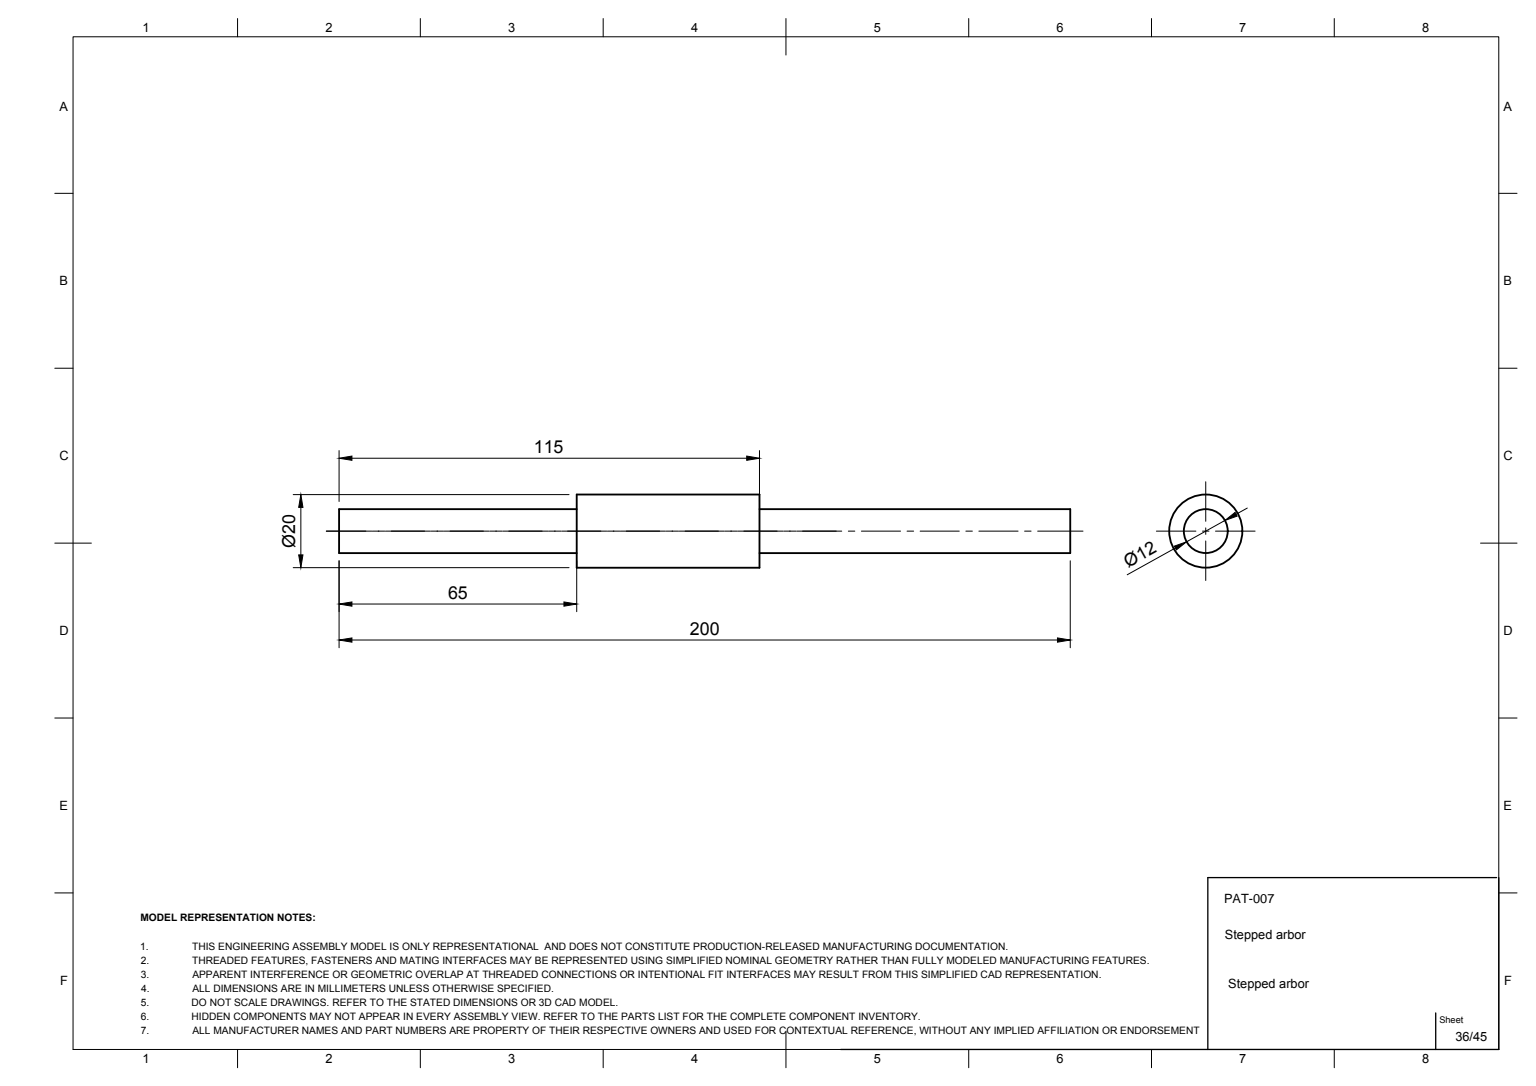
ISO-10303-21;
HEADER;
/* Generated by software containing ST-Developer
 * from STEP Tools, Inc. (www.steptools.com) 
 */

FILE_DESCRIPTION(
/* description */ ('Bearing friction torque test rig'),
/* implementation_level */ '2;1');

FILE_NAME(
/* name */ 'Stepped arbor.step',
/* time_stamp */ '2026-10-28T03:24:04-07:00',
/* author */ (''),
/* organization */ (''),
/* preprocessor_version */ 'ST-DEVELOPER v20.2',
/* originating_system */ 'Autodesk Translation Framework v15.17.0.0',
/* authorisation */ '');

FILE_SCHEMA (('AUTOMOTIVE_DESIGN { 1 0 10303 214 3 1 1 }'));
ENDSEC;

DATA;
#10=MECHANICAL_DESIGN_GEOMETRIC_PRESENTATION_REPRESENTATION('',(#582),#14822);
#489=SHAPE_REPRESENTATION_RELATIONSHIP('SRR','None',#15031,#528);
#528=ADVANCED_BREP_SHAPE_REPRESENTATION('',(#633),#14811);
#582=STYLED_ITEM('',(#15277),#633);
#633=MANIFOLD_SOLID_BREP('Body1',#7701);
#834=FACE_BOUND('',#2109,.T.);
#835=FACE_BOUND('',#2111,.T.);
#1057=PLANE('',#8995);
#1058=PLANE('',#8999);
#1059=PLANE('',#9003);
#1060=PLANE('',#9004);
#1468=FACE_OUTER_BOUND('',#2103,.T.);
#1469=FACE_OUTER_BOUND('',#2104,.T.);
#1470=FACE_OUTER_BOUND('',#2105,.T.);
#1471=FACE_OUTER_BOUND('',#2106,.T.);
#1472=FACE_OUTER_BOUND('',#2107,.T.);
#1473=FACE_OUTER_BOUND('',#2108,.T.);
#1474=FACE_OUTER_BOUND('',#2110,.T.);
#2103=EDGE_LOOP('',(#6738,#6739,#6740,#6741));
#2104=EDGE_LOOP('',(#6742));
#2105=EDGE_LOOP('',(#6743,#6744,#6745,#6746));
#2106=EDGE_LOOP('',(#6747));
#2107=EDGE_LOOP('',(#6748,#6749,#6750,#6751));
#2108=EDGE_LOOP('',(#6752));
#2109=EDGE_LOOP('',(#6753));
#2110=EDGE_LOOP('',(#6754));
#2111=EDGE_LOOP('',(#6755));
#2601=LINE('',#14102,#3045);
#2602=LINE('',#14109,#3046);
#2603=LINE('',#14116,#3047);
#3045=VECTOR('',#11252,0.6);
#3046=VECTOR('',#11261,0.6);
#3047=VECTOR('',#11270,1.);
#3482=CIRCLE('',#8993,0.6);
#3483=CIRCLE('',#8994,0.6);
#3484=CIRCLE('',#8997,0.6);
#3485=CIRCLE('',#8998,0.6);
#3486=CIRCLE('',#9001,1.);
#3487=CIRCLE('',#9002,1.);
#4097=VERTEX_POINT('',#14099);
#4098=VERTEX_POINT('',#14101);
#4099=VERTEX_POINT('',#14106);
#4100=VERTEX_POINT('',#14108);
#4101=VERTEX_POINT('',#14113);
#4102=VERTEX_POINT('',#14115);
#4995=EDGE_CURVE('',#4097,#4097,#3482,.T.);
#4996=EDGE_CURVE('',#4097,#4098,#2601,.T.);
#4997=EDGE_CURVE('',#4098,#4098,#3483,.T.);
#4998=EDGE_CURVE('',#4099,#4099,#3484,.T.);
#4999=EDGE_CURVE('',#4099,#4100,#2602,.T.);
#5000=EDGE_CURVE('',#4100,#4100,#3485,.T.);
#5001=EDGE_CURVE('',#4101,#4101,#3486,.T.);
#5002=EDGE_CURVE('',#4101,#4102,#2603,.T.);
#5003=EDGE_CURVE('',#4102,#4102,#3487,.T.);
#6738=ORIENTED_EDGE('',*,*,#4995,.F.);
#6739=ORIENTED_EDGE('',*,*,#4996,.T.);
#6740=ORIENTED_EDGE('',*,*,#4997,.F.);
#6741=ORIENTED_EDGE('',*,*,#4996,.F.);
#6742=ORIENTED_EDGE('',*,*,#4995,.T.);
#6743=ORIENTED_EDGE('',*,*,#4998,.F.);
#6744=ORIENTED_EDGE('',*,*,#4999,.T.);
#6745=ORIENTED_EDGE('',*,*,#5000,.T.);
#6746=ORIENTED_EDGE('',*,*,#4999,.F.);
#6747=ORIENTED_EDGE('',*,*,#5000,.F.);
#6748=ORIENTED_EDGE('',*,*,#5001,.F.);
#6749=ORIENTED_EDGE('',*,*,#5002,.T.);
#6750=ORIENTED_EDGE('',*,*,#5003,.T.);
#6751=ORIENTED_EDGE('',*,*,#5002,.F.);
#6752=ORIENTED_EDGE('',*,*,#5001,.T.);
#6753=ORIENTED_EDGE('',*,*,#4997,.T.);
#6754=ORIENTED_EDGE('',*,*,#5003,.F.);
#6755=ORIENTED_EDGE('',*,*,#4998,.T.);
#7178=CYLINDRICAL_SURFACE('',#8992,0.6);
#7179=CYLINDRICAL_SURFACE('',#8996,0.6);
#7180=CYLINDRICAL_SURFACE('',#9000,1.);
#7579=ADVANCED_FACE('',(#1468),#7178,.T.);
#7580=ADVANCED_FACE('',(#1469),#1057,.T.);
#7581=ADVANCED_FACE('',(#1470),#7179,.T.);
#7582=ADVANCED_FACE('',(#1471),#1058,.F.);
#7583=ADVANCED_FACE('',(#1472),#7180,.T.);
#7584=ADVANCED_FACE('',(#1473,#834),#1059,.T.);
#7585=ADVANCED_FACE('',(#1474,#835),#1060,.F.);
#7701=CLOSED_SHELL('',(#7579,#7580,#7581,#7582,#7583,#7584,#7585));
#8991=AXIS2_PLACEMENT_3D('',#14097,#11246,#11247);
#8992=AXIS2_PLACEMENT_3D('',#14098,#11248,#11249);
#8993=AXIS2_PLACEMENT_3D('',#14100,#11250,#11251);
#8994=AXIS2_PLACEMENT_3D('',#14103,#11253,#11254);
#8995=AXIS2_PLACEMENT_3D('',#14104,#11255,#11256);
#8996=AXIS2_PLACEMENT_3D('',#14105,#11257,#11258);
#8997=AXIS2_PLACEMENT_3D('',#14107,#11259,#11260);
#8998=AXIS2_PLACEMENT_3D('',#14110,#11262,#11263);
#8999=AXIS2_PLACEMENT_3D('',#14111,#11264,#11265);
#9000=AXIS2_PLACEMENT_3D('',#14112,#11266,#11267);
#9001=AXIS2_PLACEMENT_3D('',#14114,#11268,#11269);
#9002=AXIS2_PLACEMENT_3D('',#14117,#11271,#11272);
#9003=AXIS2_PLACEMENT_3D('',#14118,#11273,#11274);
#9004=AXIS2_PLACEMENT_3D('',#14119,#11275,#11276);
#11246=DIRECTION('axis',(0.,0.,1.));
#11247=DIRECTION('refdir',(1.,0.,0.));
#11248=DIRECTION('center_axis',(0.,1.,0.));
#11249=DIRECTION('ref_axis',(1.,0.,0.));
#11250=DIRECTION('center_axis',(0.,1.,0.));
#11251=DIRECTION('ref_axis',(1.,0.,0.));
#11252=DIRECTION('',(0.,-1.,0.));
#11253=DIRECTION('center_axis',(0.,-1.,0.));
#11254=DIRECTION('ref_axis',(1.,0.,0.));
#11255=DIRECTION('center_axis',(0.,1.,0.));
#11256=DIRECTION('ref_axis',(1.,0.,0.));
#11257=DIRECTION('center_axis',(0.,1.,0.));
#11258=DIRECTION('ref_axis',(1.,0.,0.));
#11259=DIRECTION('center_axis',(0.,1.,0.));
#11260=DIRECTION('ref_axis',(1.,0.,0.));
#11261=DIRECTION('',(0.,-1.,0.));
#11262=DIRECTION('center_axis',(0.,1.,0.));
#11263=DIRECTION('ref_axis',(1.,0.,0.));
#11264=DIRECTION('center_axis',(0.,1.,0.));
#11265=DIRECTION('ref_axis',(1.,0.,0.));
#11266=DIRECTION('center_axis',(0.,1.,0.));
#11267=DIRECTION('ref_axis',(1.,0.,0.));
#11268=DIRECTION('center_axis',(0.,1.,0.));
#11269=DIRECTION('ref_axis',(1.,0.,0.));
#11270=DIRECTION('',(0.,-1.,0.));
#11271=DIRECTION('center_axis',(0.,1.,0.));
#11272=DIRECTION('ref_axis',(1.,0.,0.));
#11273=DIRECTION('center_axis',(0.,1.,0.));
#11274=DIRECTION('ref_axis',(1.,0.,0.));
#11275=DIRECTION('center_axis',(0.,1.,0.));
#11276=DIRECTION('ref_axis',(1.,0.,0.));
#14097=CARTESIAN_POINT('',(0.,0.,0.));
#14098=CARTESIAN_POINT('Origin',(0.,2.5,7.));
#14099=CARTESIAN_POINT('',(-0.6,9.,7.));
#14100=CARTESIAN_POINT('Origin',(0.,9.,7.));
#14101=CARTESIAN_POINT('',(-0.6,2.5,7.));
#14102=CARTESIAN_POINT('',(-0.6,2.5,7.));
#14103=CARTESIAN_POINT('Origin',(0.,2.5,7.));
#14104=CARTESIAN_POINT('Origin',(0.,9.,7.));
#14105=CARTESIAN_POINT('Origin',(0.,-11.,7.));
#14106=CARTESIAN_POINT('',(-0.6,-2.5,7.));
#14107=CARTESIAN_POINT('Origin',(0.,-2.5,7.));
#14108=CARTESIAN_POINT('',(-0.6,-11.,7.));
#14109=CARTESIAN_POINT('',(-0.6,-11.,7.));
#14110=CARTESIAN_POINT('Origin',(0.,-11.,7.));
#14111=CARTESIAN_POINT('Origin',(0.,-11.,7.));
#14112=CARTESIAN_POINT('Origin',(0.,-2.5,7.));
#14113=CARTESIAN_POINT('',(-1.,2.5,7.));
#14114=CARTESIAN_POINT('Origin',(0.,2.5,7.));
#14115=CARTESIAN_POINT('',(-1.,-2.5,7.));
#14116=CARTESIAN_POINT('',(-1.,-2.5,7.));
#14117=CARTESIAN_POINT('Origin',(0.,-2.5,7.));
#14118=CARTESIAN_POINT('Origin',(0.,2.5,7.));
#14119=CARTESIAN_POINT('Origin',(0.,-2.5,7.));
#14766=UNCERTAINTY_MEASURE_WITH_UNIT(LENGTH_MEASURE(0.001),#14823,
'DISTANCE_ACCURACY_VALUE',
'Maximum model space distance between geometric entities at asserted c
onnectivities');
#14777=UNCERTAINTY_MEASURE_WITH_UNIT(LENGTH_MEASURE(0.001),#14823,
'DISTANCE_ACCURACY_VALUE',
'Maximum model space distance between geometric entities at asserted c
onnectivities');
#14811=(
GEOMETRIC_REPRESENTATION_CONTEXT(3)
GLOBAL_UNCERTAINTY_ASSIGNED_CONTEXT((#14766))
GLOBAL_UNIT_ASSIGNED_CONTEXT((#14823,#14825,#14826))
REPRESENTATION_CONTEXT('','3D')
);
#14822=(
GEOMETRIC_REPRESENTATION_CONTEXT(3)
GLOBAL_UNCERTAINTY_ASSIGNED_CONTEXT((#14777))
GLOBAL_UNIT_ASSIGNED_CONTEXT((#14823,#14825,#14826))
REPRESENTATION_CONTEXT('','3D')
);
#14823=(
LENGTH_UNIT()
NAMED_UNIT(*)
SI_UNIT(.CENTI.,.METRE.)
);
#14825=(
NAMED_UNIT(*)
PLANE_ANGLE_UNIT()
SI_UNIT($,.RADIAN.)
);
#14826=(
NAMED_UNIT(*)
SI_UNIT($,.STERADIAN.)
SOLID_ANGLE_UNIT()
);
#14860=SHAPE_DEFINITION_REPRESENTATION(#14970,#15031);
#14970=PRODUCT_DEFINITION_SHAPE('',$,#15076);
#15031=SHAPE_REPRESENTATION('',(#8991),#14811);
#15042=PRODUCT_DEFINITION_CONTEXT('part definition',#15176,'design');
#15076=PRODUCT_DEFINITION('Stepped arbor','Stepped arbor',#15120,#15042);
#15120=PRODUCT_DEFINITION_FORMATION('',$,#15211);
#15176=APPLICATION_CONTEXT(
'Core Data for Automotive Mechanical Design Process');
#15177=PRODUCT_CONTEXT('part definition',#15176,'mechanical');
#15211=PRODUCT('Stepped arbor','Stepped arbor','Stepped arbor',(#15177));
#15271=COLOUR_RGB('Sky Blue',0.24,0.69,0.87);
#15272=FILL_AREA_STYLE_COLOUR('',#15271);
#15273=FILL_AREA_STYLE('',(#15272));
#15274=SURFACE_STYLE_FILL_AREA(#15273);
#15275=SURFACE_SIDE_STYLE('',(#15274));
#15276=SURFACE_STYLE_USAGE(.BOTH.,#15275);
#15277=PRESENTATION_STYLE_ASSIGNMENT((#15276));
ENDSEC;
END-ISO-10303-21;
